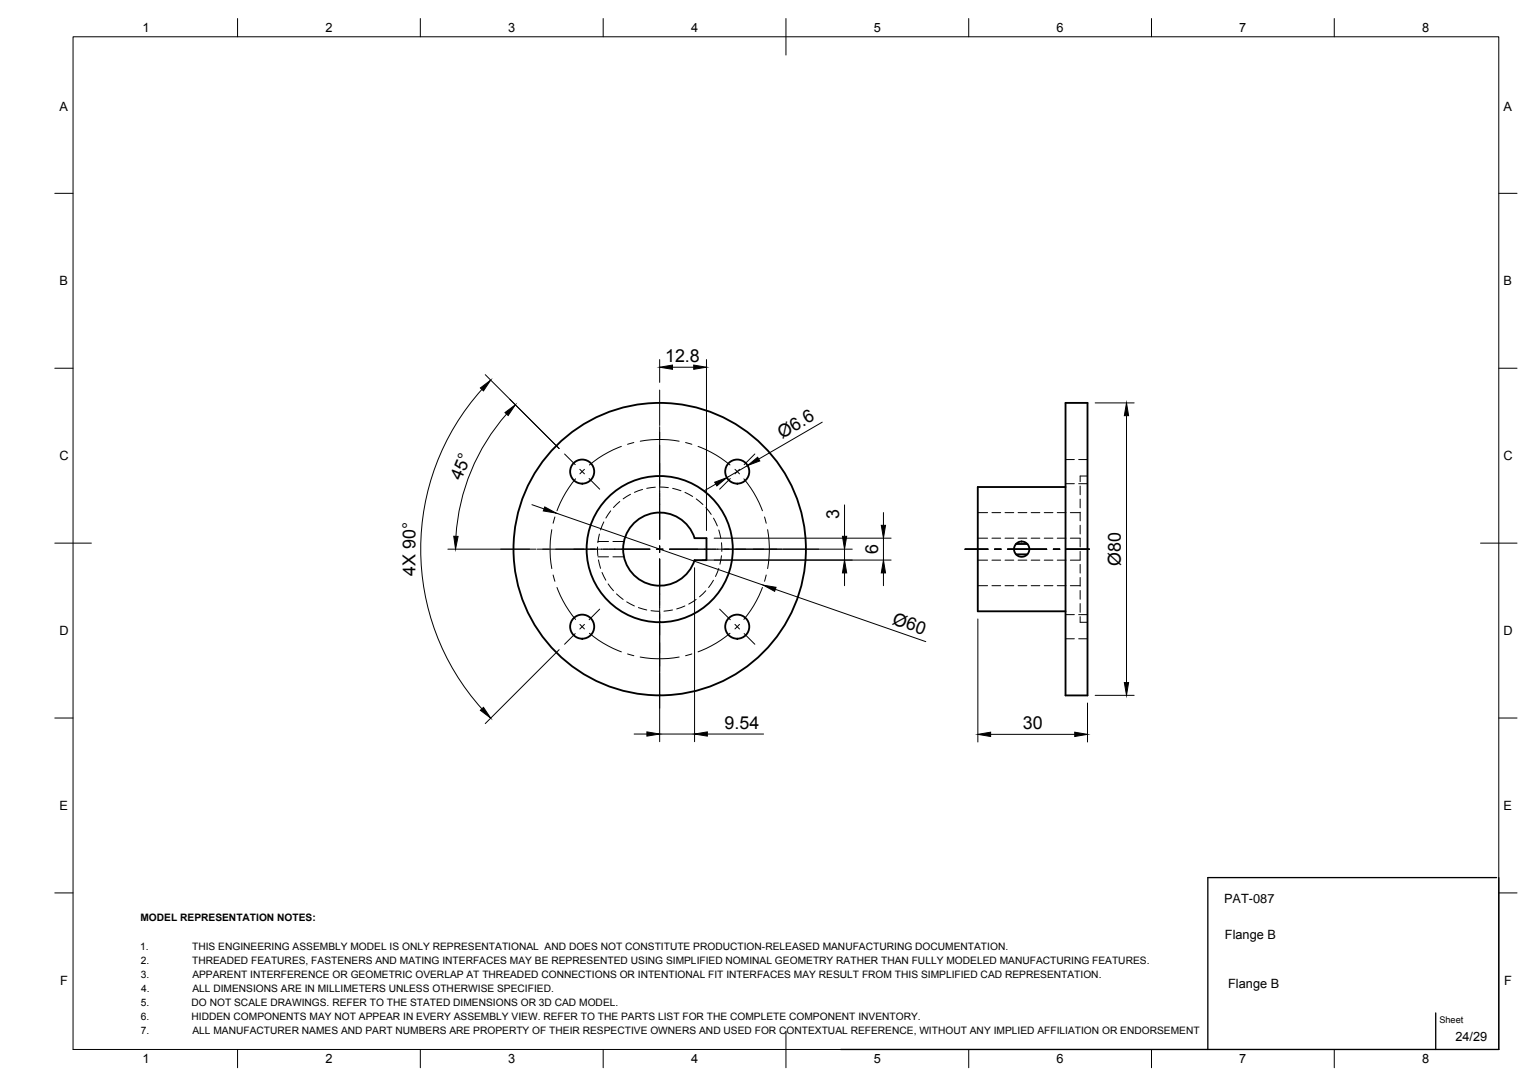
ISO-10303-21;
HEADER;
/* Generated by software containing ST-Developer
 * from STEP Tools, Inc. (www.steptools.com) 
 */

FILE_DESCRIPTION(
/* description */ ('Rigid flange shaft coupling assembly'),
/* implementation_level */ '2;1');

FILE_NAME(
/* name */ 'Flange B.step',
/* time_stamp */ '2026-10-27T10:47:16-07:00',
/* author */ (''),
/* organization */ (''),
/* preprocessor_version */ 'ST-DEVELOPER v20.2',
/* originating_system */ 'Autodesk Translation Framework v15.17.0.0',
/* authorisation */ '');

FILE_SCHEMA (('AUTOMOTIVE_DESIGN { 1 0 10303 214 3 1 1 }'));
ENDSEC;

DATA;
#10=MECHANICAL_DESIGN_GEOMETRIC_PRESENTATION_REPRESENTATION('',(#416),#9141);
#328=B_SPLINE_CURVE_WITH_KNOTS('',3,(#8346,#8347,#8348,#8349,#8350,#8351,
#8352,#8353,#8354,#8355),.UNSPECIFIED.,.F.,.F.,(4,2,2,2,4),(0.803821788694084,
0.87295099185362,0.95230721290097,1.03166343394832,1.10079263710786),
 .UNSPECIFIED.);
#329=B_SPLINE_CURVE_WITH_KNOTS('',3,(#8361,#8362,#8363,#8364,#8365,#8366,
#8367,#8368,#8369,#8370,#8371,#8372,#8373,#8374,#8375,#8376,#8377,#8378),
 .UNSPECIFIED.,.F.,.F.,(4,2,2,2,2,2,2,2,4),(0.,0.0791914196064459,0.158382839212892,
0.237573628052636,0.31676441689238,0.395955205732124,0.475145994571868,
0.554337414178314,0.63352883378476),.UNSPECIFIED.);
#330=B_SPLINE_CURVE_WITH_KNOTS('',3,(#8379,#8380,#8381,#8382,#8383,#8384,
#8385,#8386,#8387,#8388,#8389,#8390,#8391,#8392,#8393,#8394,#8395,#8396),
 .UNSPECIFIED.,.F.,.F.,(4,2,2,2,2,2,2,2,4),(0.63352883378476,0.712720253391206,
0.791911672997652,0.871102461837396,0.95029325067714,1.02948403951688,1.10867482835663,
1.18786624796307,1.26705766756952),.UNSPECIFIED.);
#331=B_SPLINE_CURVE_WITH_KNOTS('',3,(#8399,#8400,#8401,#8402,#8403,#8404,
#8405,#8406,#8407,#8408),.UNSPECIFIED.,.F.,.F.,(4,2,2,2,4),(0.168950313426773,
0.238079516586307,0.317435737633657,0.396791958681006,0.465921161840543),
 .UNSPECIFIED.);
#359=SHAPE_REPRESENTATION_RELATIONSHIP('SRR','None',#9295,#387);
#387=ADVANCED_BREP_SHAPE_REPRESENTATION('',(#444),#9130);
#416=STYLED_ITEM('',(#9486),#444);
#444=MANIFOLD_SOLID_BREP('Body1',#4771);
#537=FACE_BOUND('',#1272,.T.);
#538=FACE_BOUND('',#1274,.T.);
#539=FACE_BOUND('',#1277,.T.);
#540=FACE_BOUND('',#1278,.T.);
#541=FACE_BOUND('',#1279,.T.);
#542=FACE_BOUND('',#1280,.T.);
#543=FACE_BOUND('',#1281,.T.);
#544=FACE_BOUND('',#1284,.T.);
#545=FACE_BOUND('',#1286,.T.);
#546=FACE_BOUND('',#1288,.T.);
#547=FACE_BOUND('',#1289,.T.);
#548=FACE_BOUND('',#1290,.T.);
#549=FACE_BOUND('',#1291,.T.);
#550=FACE_BOUND('',#1292,.T.);
#672=PLANE('',#5402);
#673=PLANE('',#5407);
#674=PLANE('',#5408);
#675=PLANE('',#5409);
#676=PLANE('',#5410);
#677=PLANE('',#5411);
#678=PLANE('',#5418);
#679=PLANE('',#5425);
#680=PLANE('',#5426);
#905=FACE_OUTER_BOUND('',#1261,.T.);
#906=FACE_OUTER_BOUND('',#1262,.T.);
#907=FACE_OUTER_BOUND('',#1263,.T.);
#908=FACE_OUTER_BOUND('',#1264,.T.);
#909=FACE_OUTER_BOUND('',#1265,.T.);
#910=FACE_OUTER_BOUND('',#1266,.T.);
#911=FACE_OUTER_BOUND('',#1267,.T.);
#912=FACE_OUTER_BOUND('',#1268,.T.);
#913=FACE_OUTER_BOUND('',#1269,.T.);
#914=FACE_OUTER_BOUND('',#1270,.T.);
#915=FACE_OUTER_BOUND('',#1271,.T.);
#916=FACE_OUTER_BOUND('',#1273,.T.);
#917=FACE_OUTER_BOUND('',#1275,.T.);
#918=FACE_OUTER_BOUND('',#1276,.T.);
#919=FACE_OUTER_BOUND('',#1282,.T.);
#920=FACE_OUTER_BOUND('',#1283,.T.);
#921=FACE_OUTER_BOUND('',#1285,.T.);
#922=FACE_OUTER_BOUND('',#1287,.T.);
#1261=EDGE_LOOP('',(#3937,#3938,#3939,#3940));
#1262=EDGE_LOOP('',(#3941,#3942,#3943,#3944));
#1263=EDGE_LOOP('',(#3945,#3946,#3947,#3948));
#1264=EDGE_LOOP('',(#3949,#3950,#3951,#3952));
#1265=EDGE_LOOP('',(#3953,#3954));
#1266=EDGE_LOOP('',(#3955,#3956,#3957,#3958,#3959,#3960,#3961,#3962,#3963));
#1267=EDGE_LOOP('',(#3964,#3965,#3966));
#1268=EDGE_LOOP('',(#3967,#3968,#3969,#3970));
#1269=EDGE_LOOP('',(#3971,#3972,#3973,#3974));
#1270=EDGE_LOOP('',(#3975,#3976,#3977,#3978));
#1271=EDGE_LOOP('',(#3979));
#1272=EDGE_LOOP('',(#3980,#3981,#3982,#3983));
#1273=EDGE_LOOP('',(#3984,#3985,#3986,#3987));
#1274=EDGE_LOOP('',(#3988,#3989,#3990,#3991));
#1275=EDGE_LOOP('',(#3992,#3993,#3994,#3995));
#1276=EDGE_LOOP('',(#3996));
#1277=EDGE_LOOP('',(#3997));
#1278=EDGE_LOOP('',(#3998));
#1279=EDGE_LOOP('',(#3999));
#1280=EDGE_LOOP('',(#4000));
#1281=EDGE_LOOP('',(#4001));
#1282=EDGE_LOOP('',(#4002,#4003,#4004,#4005));
#1283=EDGE_LOOP('',(#4006,#4007,#4008,#4009));
#1284=EDGE_LOOP('',(#4010,#4011));
#1285=EDGE_LOOP('',(#4012));
#1286=EDGE_LOOP('',(#4013,#4014,#4015,#4016));
#1287=EDGE_LOOP('',(#4017));
#1288=EDGE_LOOP('',(#4018));
#1289=EDGE_LOOP('',(#4019));
#1290=EDGE_LOOP('',(#4020));
#1291=EDGE_LOOP('',(#4021));
#1292=EDGE_LOOP('',(#4022));
#1612=LINE('',#8319,#1957);
#1613=LINE('',#8325,#1958);
#1614=LINE('',#8331,#1959);
#1615=LINE('',#8337,#1960);
#1616=LINE('',#8342,#1961);
#1617=LINE('',#8359,#1962);
#1618=LINE('',#8410,#1963);
#1619=LINE('',#8414,#1964);
#1620=LINE('',#8416,#1965);
#1621=LINE('',#8418,#1966);
#1622=LINE('',#8419,#1967);
#1623=LINE('',#8423,#1968);
#1624=LINE('',#8425,#1969);
#1625=LINE('',#8427,#1970);
#1626=LINE('',#8428,#1971);
#1627=LINE('',#8430,#1972);
#1628=LINE('',#8431,#1973);
#1629=LINE('',#8441,#1974);
#1630=LINE('',#8449,#1975);
#1631=LINE('',#8454,#1976);
#1957=VECTOR('',#6447,0.33);
#1958=VECTOR('',#6454,0.33);
#1959=VECTOR('',#6461,0.33);
#1960=VECTOR('',#6468,0.33);
#1961=VECTOR('',#6473,1.);
#1962=VECTOR('',#6480,0.21);
#1963=VECTOR('',#6485,1.);
#1964=VECTOR('',#6488,1.);
#1965=VECTOR('',#6489,1.);
#1966=VECTOR('',#6490,1.);
#1967=VECTOR('',#6491,1.);
#1968=VECTOR('',#6494,1.);
#1969=VECTOR('',#6495,1.);
#1970=VECTOR('',#6496,1.);
#1971=VECTOR('',#6497,1.);
#1972=VECTOR('',#6500,1.);
#1973=VECTOR('',#6501,1.);
#1974=VECTOR('',#6516,2.);
#1975=VECTOR('',#6525,4.);
#1976=VECTOR('',#6532,1.7);
#2207=CIRCLE('',#5391,0.33);
#2208=CIRCLE('',#5392,0.33);
#2209=CIRCLE('',#5394,0.33);
#2210=CIRCLE('',#5395,0.33);
#2211=CIRCLE('',#5397,0.33);
#2212=CIRCLE('',#5398,0.33);
#2213=CIRCLE('',#5400,0.33);
#2214=CIRCLE('',#5401,0.33);
#2215=CIRCLE('',#5403,0.21);
#2216=CIRCLE('',#5405,0.21);
#2217=CIRCLE('',#5406,0.21);
#2218=CIRCLE('',#5412,2.);
#2219=CIRCLE('',#5413,1.);
#2220=CIRCLE('',#5415,1.);
#2221=CIRCLE('',#5417,2.);
#2222=CIRCLE('',#5419,4.);
#2223=CIRCLE('',#5420,1.7);
#2224=CIRCLE('',#5422,4.);
#2225=CIRCLE('',#5424,1.7);
#2514=VERTEX_POINT('',#8316);
#2515=VERTEX_POINT('',#8318);
#2516=VERTEX_POINT('',#8322);
#2517=VERTEX_POINT('',#8324);
#2518=VERTEX_POINT('',#8328);
#2519=VERTEX_POINT('',#8330);
#2520=VERTEX_POINT('',#8334);
#2521=VERTEX_POINT('',#8336);
#2522=VERTEX_POINT('',#8340);
#2523=VERTEX_POINT('',#8341);
#2524=VERTEX_POINT('',#8345);
#2525=VERTEX_POINT('',#8356);
#2526=VERTEX_POINT('',#8358);
#2527=VERTEX_POINT('',#8360);
#2528=VERTEX_POINT('',#8397);
#2529=VERTEX_POINT('',#8412);
#2530=VERTEX_POINT('',#8413);
#2531=VERTEX_POINT('',#8415);
#2532=VERTEX_POINT('',#8417);
#2533=VERTEX_POINT('',#8421);
#2534=VERTEX_POINT('',#8422);
#2535=VERTEX_POINT('',#8424);
#2536=VERTEX_POINT('',#8426);
#2537=VERTEX_POINT('',#8433);
#2538=VERTEX_POINT('',#8439);
#2539=VERTEX_POINT('',#8443);
#2540=VERTEX_POINT('',#8445);
#2541=VERTEX_POINT('',#8448);
#2542=VERTEX_POINT('',#8452);
#3012=EDGE_CURVE('',#2514,#2514,#2207,.T.);
#3013=EDGE_CURVE('',#2514,#2515,#1612,.T.);
#3014=EDGE_CURVE('',#2515,#2515,#2208,.T.);
#3015=EDGE_CURVE('',#2516,#2516,#2209,.T.);
#3016=EDGE_CURVE('',#2516,#2517,#1613,.T.);
#3017=EDGE_CURVE('',#2517,#2517,#2210,.T.);
#3018=EDGE_CURVE('',#2518,#2518,#2211,.T.);
#3019=EDGE_CURVE('',#2518,#2519,#1614,.T.);
#3020=EDGE_CURVE('',#2519,#2519,#2212,.T.);
#3021=EDGE_CURVE('',#2520,#2520,#2213,.T.);
#3022=EDGE_CURVE('',#2520,#2521,#1615,.T.);
#3023=EDGE_CURVE('',#2521,#2521,#2214,.T.);
#3024=EDGE_CURVE('',#2522,#2523,#1616,.T.);
#3025=EDGE_CURVE('',#2522,#2523,#2215,.T.);
#3026=EDGE_CURVE('',#2524,#2522,#328,.T.);
#3027=EDGE_CURVE('',#2525,#2524,#2216,.T.);
#3028=EDGE_CURVE('',#2525,#2526,#1617,.T.);
#3029=EDGE_CURVE('',#2527,#2526,#329,.T.);
#3030=EDGE_CURVE('',#2526,#2527,#330,.T.);
#3031=EDGE_CURVE('',#2528,#2525,#2217,.T.);
#3032=EDGE_CURVE('',#2523,#2528,#331,.T.);
#3033=EDGE_CURVE('',#2528,#2524,#1618,.T.);
#3034=EDGE_CURVE('',#2529,#2530,#1619,.T.);
#3035=EDGE_CURVE('',#2531,#2529,#1620,.T.);
#3036=EDGE_CURVE('',#2532,#2531,#1621,.T.);
#3037=EDGE_CURVE('',#2530,#2532,#1622,.T.);
#3038=EDGE_CURVE('',#2533,#2534,#1623,.T.);
#3039=EDGE_CURVE('',#2535,#2533,#1624,.T.);
#3040=EDGE_CURVE('',#2536,#2535,#1625,.T.);
#3041=EDGE_CURVE('',#2536,#2534,#1626,.T.);
#3042=EDGE_CURVE('',#2534,#2529,#1627,.T.);
#3043=EDGE_CURVE('',#2531,#2536,#1628,.T.);
#3044=EDGE_CURVE('',#2537,#2537,#2218,.T.);
#3045=EDGE_CURVE('',#2532,#2535,#2219,.T.);
#3046=EDGE_CURVE('',#2530,#2533,#2220,.T.);
#3047=EDGE_CURVE('',#2538,#2538,#2221,.T.);
#3048=EDGE_CURVE('',#2538,#2537,#1629,.T.);
#3049=EDGE_CURVE('',#2539,#2539,#2222,.T.);
#3050=EDGE_CURVE('',#2540,#2540,#2223,.T.);
#3051=EDGE_CURVE('',#2539,#2541,#1630,.T.);
#3052=EDGE_CURVE('',#2541,#2541,#2224,.T.);
#3053=EDGE_CURVE('',#2542,#2542,#2225,.T.);
#3054=EDGE_CURVE('',#2542,#2540,#1631,.T.);
#3937=ORIENTED_EDGE('',*,*,#3012,.F.);
#3938=ORIENTED_EDGE('',*,*,#3013,.T.);
#3939=ORIENTED_EDGE('',*,*,#3014,.F.);
#3940=ORIENTED_EDGE('',*,*,#3013,.F.);
#3941=ORIENTED_EDGE('',*,*,#3015,.F.);
#3942=ORIENTED_EDGE('',*,*,#3016,.T.);
#3943=ORIENTED_EDGE('',*,*,#3017,.F.);
#3944=ORIENTED_EDGE('',*,*,#3016,.F.);
#3945=ORIENTED_EDGE('',*,*,#3018,.F.);
#3946=ORIENTED_EDGE('',*,*,#3019,.T.);
#3947=ORIENTED_EDGE('',*,*,#3020,.F.);
#3948=ORIENTED_EDGE('',*,*,#3019,.F.);
#3949=ORIENTED_EDGE('',*,*,#3021,.F.);
#3950=ORIENTED_EDGE('',*,*,#3022,.T.);
#3951=ORIENTED_EDGE('',*,*,#3023,.F.);
#3952=ORIENTED_EDGE('',*,*,#3022,.F.);
#3953=ORIENTED_EDGE('',*,*,#3024,.F.);
#3954=ORIENTED_EDGE('',*,*,#3025,.T.);
#3955=ORIENTED_EDGE('',*,*,#3026,.F.);
#3956=ORIENTED_EDGE('',*,*,#3027,.F.);
#3957=ORIENTED_EDGE('',*,*,#3028,.T.);
#3958=ORIENTED_EDGE('',*,*,#3029,.F.);
#3959=ORIENTED_EDGE('',*,*,#3030,.F.);
#3960=ORIENTED_EDGE('',*,*,#3028,.F.);
#3961=ORIENTED_EDGE('',*,*,#3031,.F.);
#3962=ORIENTED_EDGE('',*,*,#3032,.F.);
#3963=ORIENTED_EDGE('',*,*,#3025,.F.);
#3964=ORIENTED_EDGE('',*,*,#3033,.F.);
#3965=ORIENTED_EDGE('',*,*,#3031,.T.);
#3966=ORIENTED_EDGE('',*,*,#3027,.T.);
#3967=ORIENTED_EDGE('',*,*,#3034,.F.);
#3968=ORIENTED_EDGE('',*,*,#3035,.F.);
#3969=ORIENTED_EDGE('',*,*,#3036,.F.);
#3970=ORIENTED_EDGE('',*,*,#3037,.F.);
#3971=ORIENTED_EDGE('',*,*,#3038,.F.);
#3972=ORIENTED_EDGE('',*,*,#3039,.F.);
#3973=ORIENTED_EDGE('',*,*,#3040,.F.);
#3974=ORIENTED_EDGE('',*,*,#3041,.T.);
#3975=ORIENTED_EDGE('',*,*,#3042,.F.);
#3976=ORIENTED_EDGE('',*,*,#3041,.F.);
#3977=ORIENTED_EDGE('',*,*,#3043,.F.);
#3978=ORIENTED_EDGE('',*,*,#3035,.T.);
#3979=ORIENTED_EDGE('',*,*,#3044,.F.);
#3980=ORIENTED_EDGE('',*,*,#3036,.T.);
#3981=ORIENTED_EDGE('',*,*,#3043,.T.);
#3982=ORIENTED_EDGE('',*,*,#3040,.T.);
#3983=ORIENTED_EDGE('',*,*,#3045,.F.);
#3984=ORIENTED_EDGE('',*,*,#3037,.T.);
#3985=ORIENTED_EDGE('',*,*,#3045,.T.);
#3986=ORIENTED_EDGE('',*,*,#3039,.T.);
#3987=ORIENTED_EDGE('',*,*,#3046,.F.);
#3988=ORIENTED_EDGE('',*,*,#3032,.T.);
#3989=ORIENTED_EDGE('',*,*,#3033,.T.);
#3990=ORIENTED_EDGE('',*,*,#3026,.T.);
#3991=ORIENTED_EDGE('',*,*,#3024,.T.);
#3992=ORIENTED_EDGE('',*,*,#3047,.F.);
#3993=ORIENTED_EDGE('',*,*,#3048,.T.);
#3994=ORIENTED_EDGE('',*,*,#3044,.T.);
#3995=ORIENTED_EDGE('',*,*,#3048,.F.);
#3996=ORIENTED_EDGE('',*,*,#3049,.T.);
#3997=ORIENTED_EDGE('',*,*,#3050,.F.);
#3998=ORIENTED_EDGE('',*,*,#3023,.T.);
#3999=ORIENTED_EDGE('',*,*,#3020,.T.);
#4000=ORIENTED_EDGE('',*,*,#3017,.T.);
#4001=ORIENTED_EDGE('',*,*,#3014,.T.);
#4002=ORIENTED_EDGE('',*,*,#3049,.F.);
#4003=ORIENTED_EDGE('',*,*,#3051,.T.);
#4004=ORIENTED_EDGE('',*,*,#3052,.T.);
#4005=ORIENTED_EDGE('',*,*,#3051,.F.);
#4006=ORIENTED_EDGE('',*,*,#3053,.F.);
#4007=ORIENTED_EDGE('',*,*,#3054,.T.);
#4008=ORIENTED_EDGE('',*,*,#3050,.T.);
#4009=ORIENTED_EDGE('',*,*,#3054,.F.);
#4010=ORIENTED_EDGE('',*,*,#3029,.T.);
#4011=ORIENTED_EDGE('',*,*,#3030,.T.);
#4012=ORIENTED_EDGE('',*,*,#3053,.T.);
#4013=ORIENTED_EDGE('',*,*,#3034,.T.);
#4014=ORIENTED_EDGE('',*,*,#3046,.T.);
#4015=ORIENTED_EDGE('',*,*,#3038,.T.);
#4016=ORIENTED_EDGE('',*,*,#3042,.T.);
#4017=ORIENTED_EDGE('',*,*,#3052,.F.);
#4018=ORIENTED_EDGE('',*,*,#3047,.T.);
#4019=ORIENTED_EDGE('',*,*,#3021,.T.);
#4020=ORIENTED_EDGE('',*,*,#3018,.T.);
#4021=ORIENTED_EDGE('',*,*,#3015,.T.);
#4022=ORIENTED_EDGE('',*,*,#3012,.T.);
#4453=CYLINDRICAL_SURFACE('',#5390,0.33);
#4454=CYLINDRICAL_SURFACE('',#5393,0.33);
#4455=CYLINDRICAL_SURFACE('',#5396,0.33);
#4456=CYLINDRICAL_SURFACE('',#5399,0.33);
#4457=CYLINDRICAL_SURFACE('',#5404,0.21);
#4458=CYLINDRICAL_SURFACE('',#5414,1.);
#4459=CYLINDRICAL_SURFACE('',#5416,2.);
#4460=CYLINDRICAL_SURFACE('',#5421,4.);
#4461=CYLINDRICAL_SURFACE('',#5423,1.7);
#4641=ADVANCED_FACE('',(#905),#4453,.F.);
#4642=ADVANCED_FACE('',(#906),#4454,.F.);
#4643=ADVANCED_FACE('',(#907),#4455,.F.);
#4644=ADVANCED_FACE('',(#908),#4456,.F.);
#4645=ADVANCED_FACE('',(#909),#672,.T.);
#4646=ADVANCED_FACE('',(#910),#4457,.F.);
#4647=ADVANCED_FACE('',(#911),#673,.T.);
#4648=ADVANCED_FACE('',(#912),#674,.F.);
#4649=ADVANCED_FACE('',(#913),#675,.F.);
#4650=ADVANCED_FACE('',(#914),#676,.F.);
#4651=ADVANCED_FACE('',(#915,#537),#677,.F.);
#4652=ADVANCED_FACE('',(#916,#538),#4458,.F.);
#4653=ADVANCED_FACE('',(#917),#4459,.F.);
#4654=ADVANCED_FACE('',(#918,#539,#540,#541,#542,#543),#678,.T.);
#4655=ADVANCED_FACE('',(#919),#4460,.T.);
#4656=ADVANCED_FACE('',(#920,#544),#4461,.T.);
#4657=ADVANCED_FACE('',(#921,#545),#679,.T.);
#4658=ADVANCED_FACE('',(#922,#546,#547,#548,#549,#550),#680,.F.);
#4771=CLOSED_SHELL('',(#4641,#4642,#4643,#4644,#4645,#4646,#4647,#4648,
#4649,#4650,#4651,#4652,#4653,#4654,#4655,#4656,#4657,#4658));
#5389=AXIS2_PLACEMENT_3D('',#8314,#6441,#6442);
#5390=AXIS2_PLACEMENT_3D('',#8315,#6443,#6444);
#5391=AXIS2_PLACEMENT_3D('',#8317,#6445,#6446);
#5392=AXIS2_PLACEMENT_3D('',#8320,#6448,#6449);
#5393=AXIS2_PLACEMENT_3D('',#8321,#6450,#6451);
#5394=AXIS2_PLACEMENT_3D('',#8323,#6452,#6453);
#5395=AXIS2_PLACEMENT_3D('',#8326,#6455,#6456);
#5396=AXIS2_PLACEMENT_3D('',#8327,#6457,#6458);
#5397=AXIS2_PLACEMENT_3D('',#8329,#6459,#6460);
#5398=AXIS2_PLACEMENT_3D('',#8332,#6462,#6463);
#5399=AXIS2_PLACEMENT_3D('',#8333,#6464,#6465);
#5400=AXIS2_PLACEMENT_3D('',#8335,#6466,#6467);
#5401=AXIS2_PLACEMENT_3D('',#8338,#6469,#6470);
#5402=AXIS2_PLACEMENT_3D('',#8339,#6471,#6472);
#5403=AXIS2_PLACEMENT_3D('',#8343,#6474,#6475);
#5404=AXIS2_PLACEMENT_3D('',#8344,#6476,#6477);
#5405=AXIS2_PLACEMENT_3D('',#8357,#6478,#6479);
#5406=AXIS2_PLACEMENT_3D('',#8398,#6481,#6482);
#5407=AXIS2_PLACEMENT_3D('',#8409,#6483,#6484);
#5408=AXIS2_PLACEMENT_3D('',#8411,#6486,#6487);
#5409=AXIS2_PLACEMENT_3D('',#8420,#6492,#6493);
#5410=AXIS2_PLACEMENT_3D('',#8429,#6498,#6499);
#5411=AXIS2_PLACEMENT_3D('',#8432,#6502,#6503);
#5412=AXIS2_PLACEMENT_3D('',#8434,#6504,#6505);
#5413=AXIS2_PLACEMENT_3D('',#8435,#6506,#6507);
#5414=AXIS2_PLACEMENT_3D('',#8436,#6508,#6509);
#5415=AXIS2_PLACEMENT_3D('',#8437,#6510,#6511);
#5416=AXIS2_PLACEMENT_3D('',#8438,#6512,#6513);
#5417=AXIS2_PLACEMENT_3D('',#8440,#6514,#6515);
#5418=AXIS2_PLACEMENT_3D('',#8442,#6517,#6518);
#5419=AXIS2_PLACEMENT_3D('',#8444,#6519,#6520);
#5420=AXIS2_PLACEMENT_3D('',#8446,#6521,#6522);
#5421=AXIS2_PLACEMENT_3D('',#8447,#6523,#6524);
#5422=AXIS2_PLACEMENT_3D('',#8450,#6526,#6527);
#5423=AXIS2_PLACEMENT_3D('',#8451,#6528,#6529);
#5424=AXIS2_PLACEMENT_3D('',#8453,#6530,#6531);
#5425=AXIS2_PLACEMENT_3D('',#8455,#6533,#6534);
#5426=AXIS2_PLACEMENT_3D('',#8456,#6535,#6536);
#6441=DIRECTION('axis',(0.,0.,1.));
#6442=DIRECTION('refdir',(1.,0.,0.));
#6443=DIRECTION('center_axis',(0.,1.,0.));
#6444=DIRECTION('ref_axis',(1.,0.,0.));
#6445=DIRECTION('center_axis',(0.,1.,0.));
#6446=DIRECTION('ref_axis',(1.,0.,0.));
#6447=DIRECTION('',(0.,1.,0.));
#6448=DIRECTION('center_axis',(0.,-1.,0.));
#6449=DIRECTION('ref_axis',(1.,0.,0.));
#6450=DIRECTION('center_axis',(0.,1.,0.));
#6451=DIRECTION('ref_axis',(1.,0.,0.));
#6452=DIRECTION('center_axis',(0.,1.,0.));
#6453=DIRECTION('ref_axis',(1.,0.,0.));
#6454=DIRECTION('',(0.,1.,0.));
#6455=DIRECTION('center_axis',(0.,-1.,0.));
#6456=DIRECTION('ref_axis',(1.,0.,0.));
#6457=DIRECTION('center_axis',(0.,1.,0.));
#6458=DIRECTION('ref_axis',(1.,0.,0.));
#6459=DIRECTION('center_axis',(0.,1.,0.));
#6460=DIRECTION('ref_axis',(1.,0.,0.));
#6461=DIRECTION('',(0.,1.,0.));
#6462=DIRECTION('center_axis',(0.,-1.,0.));
#6463=DIRECTION('ref_axis',(1.,0.,0.));
#6464=DIRECTION('center_axis',(0.,1.,0.));
#6465=DIRECTION('ref_axis',(1.,0.,0.));
#6466=DIRECTION('center_axis',(0.,1.,0.));
#6467=DIRECTION('ref_axis',(1.,0.,0.));
#6468=DIRECTION('',(0.,1.,0.));
#6469=DIRECTION('center_axis',(0.,-1.,0.));
#6470=DIRECTION('ref_axis',(1.,0.,0.));
#6471=DIRECTION('center_axis',(0.,0.,1.));
#6472=DIRECTION('ref_axis',(1.,0.,0.));
#6473=DIRECTION('',(0.,1.,0.));
#6474=DIRECTION('center_axis',(0.,0.,1.));
#6475=DIRECTION('ref_axis',(1.,0.,0.));
#6476=DIRECTION('center_axis',(0.,0.,1.));
#6477=DIRECTION('ref_axis',(1.,0.,0.));
#6478=DIRECTION('center_axis',(0.,0.,1.));
#6479=DIRECTION('ref_axis',(1.,0.,0.));
#6480=DIRECTION('',(0.,0.,1.));
#6481=DIRECTION('center_axis',(0.,0.,1.));
#6482=DIRECTION('ref_axis',(1.,0.,0.));
#6483=DIRECTION('center_axis',(0.,0.,1.));
#6484=DIRECTION('ref_axis',(1.,0.,0.));
#6485=DIRECTION('',(0.,-1.,0.));
#6486=DIRECTION('center_axis',(1.,0.,0.));
#6487=DIRECTION('ref_axis',(0.,0.,-1.));
#6488=DIRECTION('',(0.,0.,1.));
#6489=DIRECTION('',(0.,1.,0.));
#6490=DIRECTION('',(0.,0.,-1.));
#6491=DIRECTION('',(0.,-1.,0.));
#6492=DIRECTION('center_axis',(-1.,0.,0.));
#6493=DIRECTION('ref_axis',(0.,0.,1.));
#6494=DIRECTION('',(0.,0.,-1.));
#6495=DIRECTION('',(0.,1.,0.));
#6496=DIRECTION('',(0.,0.,1.));
#6497=DIRECTION('',(0.,1.,0.));
#6498=DIRECTION('center_axis',(0.,0.,-1.));
#6499=DIRECTION('ref_axis',(-1.,0.,0.));
#6500=DIRECTION('',(1.,0.,0.));
#6501=DIRECTION('',(-1.,0.,0.));
#6502=DIRECTION('center_axis',(0.,1.,0.));
#6503=DIRECTION('ref_axis',(1.,0.,0.));
#6504=DIRECTION('center_axis',(0.,1.,0.));
#6505=DIRECTION('ref_axis',(1.,0.,0.));
#6506=DIRECTION('center_axis',(0.,-1.,0.));
#6507=DIRECTION('ref_axis',(1.,0.,0.));
#6508=DIRECTION('center_axis',(0.,1.,0.));
#6509=DIRECTION('ref_axis',(6.12323399573677E-17,0.,1.));
#6510=DIRECTION('center_axis',(0.,-1.,0.));
#6511=DIRECTION('ref_axis',(1.,0.,0.));
#6512=DIRECTION('center_axis',(0.,1.,0.));
#6513=DIRECTION('ref_axis',(1.,0.,0.));
#6514=DIRECTION('center_axis',(0.,1.,0.));
#6515=DIRECTION('ref_axis',(1.,0.,0.));
#6516=DIRECTION('',(0.,1.,0.));
#6517=DIRECTION('center_axis',(0.,1.,0.));
#6518=DIRECTION('ref_axis',(1.,0.,0.));
#6519=DIRECTION('center_axis',(0.,1.,0.));
#6520=DIRECTION('ref_axis',(1.,0.,0.));
#6521=DIRECTION('center_axis',(0.,1.,0.));
#6522=DIRECTION('ref_axis',(1.,0.,0.));
#6523=DIRECTION('center_axis',(0.,1.,0.));
#6524=DIRECTION('ref_axis',(1.,0.,0.));
#6525=DIRECTION('',(0.,-1.,0.));
#6526=DIRECTION('center_axis',(0.,1.,0.));
#6527=DIRECTION('ref_axis',(1.,0.,0.));
#6528=DIRECTION('center_axis',(0.,1.,0.));
#6529=DIRECTION('ref_axis',(1.,0.,0.));
#6530=DIRECTION('center_axis',(0.,1.,0.));
#6531=DIRECTION('ref_axis',(1.,0.,0.));
#6532=DIRECTION('',(0.,-1.,0.));
#6533=DIRECTION('center_axis',(0.,1.,0.));
#6534=DIRECTION('ref_axis',(1.,0.,0.));
#6535=DIRECTION('center_axis',(0.,1.,0.));
#6536=DIRECTION('ref_axis',(1.,0.,0.));
#8314=CARTESIAN_POINT('',(0.,0.,0.));
#8315=CARTESIAN_POINT('Origin',(-2.12132034355964,9.3,4.40867965644036));
#8316=CARTESIAN_POINT('',(-2.45132034355964,10.,4.40867965644036));
#8317=CARTESIAN_POINT('Origin',(-2.12132034355964,10.,4.40867965644036));
#8318=CARTESIAN_POINT('',(-2.45132034355964,10.6,4.40867965644036));
#8319=CARTESIAN_POINT('',(-2.45132034355964,9.3,4.40867965644036));
#8320=CARTESIAN_POINT('Origin',(-2.12132034355964,10.6,4.40867965644036));
#8321=CARTESIAN_POINT('Origin',(-2.12132034355964,9.3,8.65132034355964));
#8322=CARTESIAN_POINT('',(-2.45132034355964,10.,8.65132034355964));
#8323=CARTESIAN_POINT('Origin',(-2.12132034355964,10.,8.65132034355964));
#8324=CARTESIAN_POINT('',(-2.45132034355964,10.6,8.65132034355964));
#8325=CARTESIAN_POINT('',(-2.45132034355964,9.3,8.65132034355964));
#8326=CARTESIAN_POINT('Origin',(-2.12132034355964,10.6,8.65132034355964));
#8327=CARTESIAN_POINT('Origin',(2.12132034355964,9.3,8.65132034355964));
#8328=CARTESIAN_POINT('',(1.79132034355964,10.,8.65132034355964));
#8329=CARTESIAN_POINT('Origin',(2.12132034355964,10.,8.65132034355964));
#8330=CARTESIAN_POINT('',(1.79132034355964,10.6,8.65132034355964));
#8331=CARTESIAN_POINT('',(1.79132034355964,9.3,8.65132034355964));
#8332=CARTESIAN_POINT('Origin',(2.12132034355964,10.6,8.65132034355964));
#8333=CARTESIAN_POINT('Origin',(2.12132034355964,9.3,4.40867965644036));
#8334=CARTESIAN_POINT('',(1.79132034355964,10.,4.40867965644036));
#8335=CARTESIAN_POINT('Origin',(2.12132034355964,10.,4.40867965644036));
#8336=CARTESIAN_POINT('',(1.79132034355964,10.6,4.40867965644036));
#8337=CARTESIAN_POINT('',(1.79132034355964,9.3,4.40867965644036));
#8338=CARTESIAN_POINT('Origin',(2.12132034355964,10.6,4.40867965644036));
#8339=CARTESIAN_POINT('Origin',(0.,11.8,7.52));
#8340=CARTESIAN_POINT('',(0.141067359796651,11.644436508139,7.52));
#8341=CARTESIAN_POINT('',(0.141067359796651,11.955563491861,7.52));
#8342=CARTESIAN_POINT('',(0.141067359796651,10.,7.52));
#8343=CARTESIAN_POINT('Origin',(0.,11.8,7.52));
#8344=CARTESIAN_POINT('Origin',(0.,11.8,7.52));
#8345=CARTESIAN_POINT('',(-0.141067359796651,11.644436508139,7.52));
#8346=CARTESIAN_POINT('Ctrl Pts',(-0.141067359796652,11.644436508139,7.52));
#8347=CARTESIAN_POINT('Ctrl Pts',(-0.12381835669822,11.6287948476368,7.52245784982447));
#8348=CARTESIAN_POINT('Ctrl Pts',(-0.102998643109696,11.615375956669,7.52493819304946));
#8349=CARTESIAN_POINT('Ctrl Pts',(-0.0546141143983528,11.5953025362756,
7.52884449237241));
#8350=CARTESIAN_POINT('Ctrl Pts',(-0.0264520736824499,11.59,7.53));
#8351=CARTESIAN_POINT('Ctrl Pts',(0.0264520736824499,11.59,7.53));
#8352=CARTESIAN_POINT('Ctrl Pts',(0.054614114398353,11.5953025362756,7.52884449237241));
#8353=CARTESIAN_POINT('Ctrl Pts',(0.102998643109697,11.615375956669,7.52493819304946));
#8354=CARTESIAN_POINT('Ctrl Pts',(0.123818356698218,11.6287948476368,7.52245784982447));
#8355=CARTESIAN_POINT('Ctrl Pts',(0.141067359796651,11.644436508139,7.52));
#8356=CARTESIAN_POINT('',(-0.21,11.8,7.52));
#8357=CARTESIAN_POINT('Origin',(0.,11.8,7.52));
#8358=CARTESIAN_POINT('',(-0.21,11.8,8.21697954937219));
#8359=CARTESIAN_POINT('',(-0.21,11.8,7.52));
#8360=CARTESIAN_POINT('',(0.21,11.8,8.21697954937219));
#8361=CARTESIAN_POINT('Ctrl Pts',(0.21,11.8,8.21697954937219));
#8362=CARTESIAN_POINT('Ctrl Pts',(0.21,11.7736028601312,8.21697954937219));
#8363=CARTESIAN_POINT('Ctrl Pts',(0.204718998643499,11.7454648357413,8.21766304765575));
#8364=CARTESIAN_POINT('Ctrl Pts',(0.183279390356407,11.6937332670887,8.22012576310987));
#8365=CARTESIAN_POINT('Ctrl Pts',(0.167122246533942,11.6701373984356,8.22186875774124));
#8366=CARTESIAN_POINT('Ctrl Pts',(0.129862749952602,11.6328779018543,8.22513580556568));
#8367=CARTESIAN_POINT('Ctrl Pts',(0.106266816759542,11.6167206417943,8.22687297932906));
#8368=CARTESIAN_POINT('Ctrl Pts',(0.0545350296960238,11.5952809481877,8.22932235754078));
#8369=CARTESIAN_POINT('Ctrl Pts',(0.0263969296132481,11.59,8.23));
#8370=CARTESIAN_POINT('Ctrl Pts',(-0.026396929613248,11.59,8.23));
#8371=CARTESIAN_POINT('Ctrl Pts',(-0.0545350296960238,11.5952809481877,
8.22932235754078));
#8372=CARTESIAN_POINT('Ctrl Pts',(-0.106266816759542,11.6167206417943,8.22687297932906));
#8373=CARTESIAN_POINT('Ctrl Pts',(-0.129862749952602,11.6328779018543,8.22513580556568));
#8374=CARTESIAN_POINT('Ctrl Pts',(-0.167122246533941,11.6701373984356,8.22186875774124));
#8375=CARTESIAN_POINT('Ctrl Pts',(-0.183279390356407,11.6937332670887,8.22012576310987));
#8376=CARTESIAN_POINT('Ctrl Pts',(-0.204718998643499,11.7454648357413,8.21766304765575));
#8377=CARTESIAN_POINT('Ctrl Pts',(-0.21,11.7736028601312,8.21697954937219));
#8378=CARTESIAN_POINT('Ctrl Pts',(-0.21,11.8,8.21697954937219));
#8379=CARTESIAN_POINT('Ctrl Pts',(-0.21,11.8,8.21697954937219));
#8380=CARTESIAN_POINT('Ctrl Pts',(-0.21,11.8263971398688,8.21697954937219));
#8381=CARTESIAN_POINT('Ctrl Pts',(-0.204718998643499,11.8545351642587,8.21766304765575));
#8382=CARTESIAN_POINT('Ctrl Pts',(-0.183279390356407,11.9062667329113,8.22012576310987));
#8383=CARTESIAN_POINT('Ctrl Pts',(-0.167122246533942,11.9298626015644,8.22186875774124));
#8384=CARTESIAN_POINT('Ctrl Pts',(-0.129862749952602,11.9671220981457,8.22513580556568));
#8385=CARTESIAN_POINT('Ctrl Pts',(-0.106266816759542,11.9832793582057,8.22687297932906));
#8386=CARTESIAN_POINT('Ctrl Pts',(-0.0545350296960238,12.0047190518123,
8.22932235754078));
#8387=CARTESIAN_POINT('Ctrl Pts',(-0.0263969296132481,12.01,8.23));
#8388=CARTESIAN_POINT('Ctrl Pts',(0.026396929613248,12.01,8.23));
#8389=CARTESIAN_POINT('Ctrl Pts',(0.0545350296960238,12.0047190518123,8.22932235754078));
#8390=CARTESIAN_POINT('Ctrl Pts',(0.106266816759542,11.9832793582057,8.22687297932906));
#8391=CARTESIAN_POINT('Ctrl Pts',(0.129862749952602,11.9671220981457,8.22513580556568));
#8392=CARTESIAN_POINT('Ctrl Pts',(0.167122246533941,11.9298626015644,8.22186875774124));
#8393=CARTESIAN_POINT('Ctrl Pts',(0.183279390356408,11.9062667329113,8.22012576310987));
#8394=CARTESIAN_POINT('Ctrl Pts',(0.204718998643499,11.8545351642587,8.21766304765575));
#8395=CARTESIAN_POINT('Ctrl Pts',(0.21,11.8263971398688,8.21697954937219));
#8396=CARTESIAN_POINT('Ctrl Pts',(0.21,11.8,8.21697954937219));
#8397=CARTESIAN_POINT('',(-0.141067359796651,11.955563491861,7.52));
#8398=CARTESIAN_POINT('Origin',(0.,11.8,7.52));
#8399=CARTESIAN_POINT('Ctrl Pts',(0.141067359796651,11.955563491861,7.52));
#8400=CARTESIAN_POINT('Ctrl Pts',(0.123818356698221,11.9712051523632,7.52245784982447));
#8401=CARTESIAN_POINT('Ctrl Pts',(0.102998643109695,11.984624043331,7.52493819304946));
#8402=CARTESIAN_POINT('Ctrl Pts',(0.0546141143983528,12.0046974637244,7.52884449237241));
#8403=CARTESIAN_POINT('Ctrl Pts',(0.0264520736824499,12.01,7.53));
#8404=CARTESIAN_POINT('Ctrl Pts',(-0.0264520736824498,12.01,7.53));
#8405=CARTESIAN_POINT('Ctrl Pts',(-0.0546141143983515,12.0046974637244,
7.52884449237241));
#8406=CARTESIAN_POINT('Ctrl Pts',(-0.102998643109696,11.984624043331,7.52493819304946));
#8407=CARTESIAN_POINT('Ctrl Pts',(-0.123818356698219,11.9712051523632,7.52245784982447));
#8408=CARTESIAN_POINT('Ctrl Pts',(-0.14106735979665,11.955563491861,7.52));
#8409=CARTESIAN_POINT('Origin',(0.,11.8,7.52));
#8410=CARTESIAN_POINT('',(-0.141067359796651,10.,7.52));
#8411=CARTESIAN_POINT('Origin',(0.3,9.9,6.53));
#8412=CARTESIAN_POINT('',(0.3,13.,5.25));
#8413=CARTESIAN_POINT('',(0.3,13.,5.57606079858305));
#8414=CARTESIAN_POINT('',(0.3,13.,6.53));
#8415=CARTESIAN_POINT('',(0.3,10.2,5.25));
#8416=CARTESIAN_POINT('',(0.3,9.9,5.25));
#8417=CARTESIAN_POINT('',(0.3,10.2,5.57606079858305));
#8418=CARTESIAN_POINT('',(0.3,10.2,6.53));
#8419=CARTESIAN_POINT('',(0.3,10.,5.57606079858305));
#8420=CARTESIAN_POINT('Origin',(-0.3,9.9,5.25));
#8421=CARTESIAN_POINT('',(-0.3,13.,5.57606079858305));
#8422=CARTESIAN_POINT('',(-0.3,13.,5.25));
#8423=CARTESIAN_POINT('',(-0.3,13.,5.89));
#8424=CARTESIAN_POINT('',(-0.3,10.2,5.57606079858305));
#8425=CARTESIAN_POINT('',(-0.3,10.,5.57606079858305));
#8426=CARTESIAN_POINT('',(-0.3,10.2,5.25));
#8427=CARTESIAN_POINT('',(-0.3,10.2,5.89));
#8428=CARTESIAN_POINT('',(-0.3,9.9,5.25));
#8429=CARTESIAN_POINT('Origin',(0.3,9.9,5.25));
#8430=CARTESIAN_POINT('',(0.15,13.,5.25));
#8431=CARTESIAN_POINT('',(0.15,10.2,5.25));
#8432=CARTESIAN_POINT('Origin',(0.,10.2,6.53));
#8433=CARTESIAN_POINT('',(-2.,10.2,6.53));
#8434=CARTESIAN_POINT('Origin',(0.,10.2,6.53));
#8435=CARTESIAN_POINT('Origin',(0.,10.2,6.53));
#8436=CARTESIAN_POINT('Origin',(0.,10.,6.53));
#8437=CARTESIAN_POINT('Origin',(0.,13.,6.53));
#8438=CARTESIAN_POINT('Origin',(0.,9.99,6.53));
#8439=CARTESIAN_POINT('',(-2.,10.,6.53));
#8440=CARTESIAN_POINT('Origin',(0.,10.,6.53));
#8441=CARTESIAN_POINT('',(-2.,9.99,6.53));
#8442=CARTESIAN_POINT('Origin',(0.,10.6,6.53));
#8443=CARTESIAN_POINT('',(-4.,10.6,6.53));
#8444=CARTESIAN_POINT('Origin',(0.,10.6,6.53));
#8445=CARTESIAN_POINT('',(-1.7,10.6,6.53));
#8446=CARTESIAN_POINT('Origin',(0.,10.6,6.53));
#8447=CARTESIAN_POINT('Origin',(0.,10.,6.53));
#8448=CARTESIAN_POINT('',(-4.,10.,6.53));
#8449=CARTESIAN_POINT('',(-4.,10.,6.53));
#8450=CARTESIAN_POINT('Origin',(0.,10.,6.53));
#8451=CARTESIAN_POINT('Origin',(0.,10.,6.53));
#8452=CARTESIAN_POINT('',(-1.7,13.,6.53));
#8453=CARTESIAN_POINT('Origin',(0.,13.,6.53));
#8454=CARTESIAN_POINT('',(-1.7,10.,6.53));
#8455=CARTESIAN_POINT('Origin',(0.,13.,6.53));
#8456=CARTESIAN_POINT('Origin',(0.,10.,6.53));
#9097=UNCERTAINTY_MEASURE_WITH_UNIT(LENGTH_MEASURE(0.001),#9142,
'DISTANCE_ACCURACY_VALUE',
'Maximum model space distance between geometric entities at asserted c
onnectivities');
#9108=UNCERTAINTY_MEASURE_WITH_UNIT(LENGTH_MEASURE(0.001),#9142,
'DISTANCE_ACCURACY_VALUE',
'Maximum model space distance between geometric entities at asserted c
onnectivities');
#9130=(
GEOMETRIC_REPRESENTATION_CONTEXT(3)
GLOBAL_UNCERTAINTY_ASSIGNED_CONTEXT((#9097))
GLOBAL_UNIT_ASSIGNED_CONTEXT((#9142,#9144,#9145))
REPRESENTATION_CONTEXT('','3D')
);
#9141=(
GEOMETRIC_REPRESENTATION_CONTEXT(3)
GLOBAL_UNCERTAINTY_ASSIGNED_CONTEXT((#9108))
GLOBAL_UNIT_ASSIGNED_CONTEXT((#9142,#9144,#9145))
REPRESENTATION_CONTEXT('','3D')
);
#9142=(
LENGTH_UNIT()
NAMED_UNIT(*)
SI_UNIT(.CENTI.,.METRE.)
);
#9144=(
NAMED_UNIT(*)
PLANE_ANGLE_UNIT()
SI_UNIT($,.RADIAN.)
);
#9145=(
NAMED_UNIT(*)
SI_UNIT($,.STERADIAN.)
SOLID_ANGLE_UNIT()
);
#9167=SHAPE_DEFINITION_REPRESENTATION(#9201,#9295);
#9201=PRODUCT_DEFINITION_SHAPE('',$,#9328);
#9295=SHAPE_REPRESENTATION('',(#5389),#9130);
#9306=PRODUCT_DEFINITION_CONTEXT('part definition',#9404,'design');
#9328=PRODUCT_DEFINITION('Flange B','Flange B',#9360,#9306);
#9360=PRODUCT_DEFINITION_FORMATION('',$,#9427);
#9404=APPLICATION_CONTEXT(
'Core Data for Automotive Mechanical Design Process');
#9405=PRODUCT_CONTEXT('part definition',#9404,'mechanical');
#9427=PRODUCT('Flange B','Flange B','Flange B',(#9405));
#9480=COLOUR_RGB('Light Blue',0.38,0.62,0.78);
#9481=FILL_AREA_STYLE_COLOUR('',#9480);
#9482=FILL_AREA_STYLE('',(#9481));
#9483=SURFACE_STYLE_FILL_AREA(#9482);
#9484=SURFACE_SIDE_STYLE('',(#9483));
#9485=SURFACE_STYLE_USAGE(.BOTH.,#9484);
#9486=PRESENTATION_STYLE_ASSIGNMENT((#9485));
ENDSEC;
END-ISO-10303-21;
